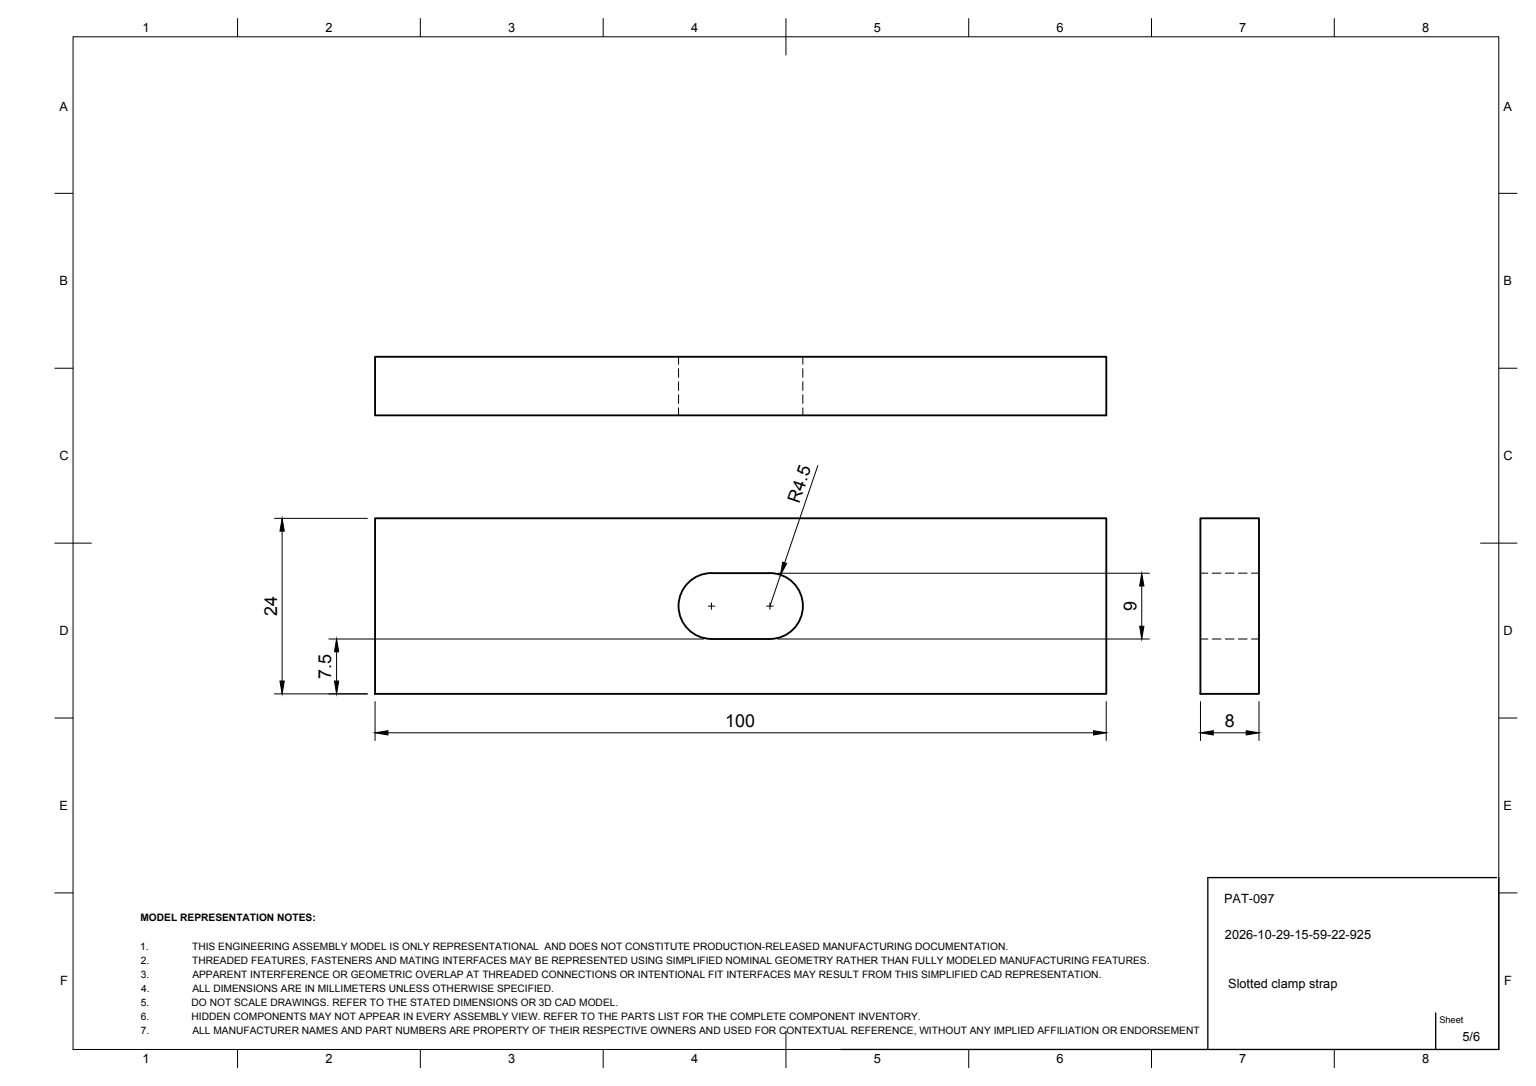
ISO-10303-21;
HEADER;
/* Generated by software containing ST-Developer
 * from STEP Tools, Inc. (www.steptools.com) 
 */

FILE_DESCRIPTION(
/* description */ ('PAT-097'),
/* implementation_level */ '2;1');

FILE_NAME(
/* name */ 'Slotted clamp strap.step',
/* time_stamp */ '2026-10-29T15:59:31-07:00',
/* author */ (''),
/* organization */ (''),
/* preprocessor_version */ 'ST-DEVELOPER v20.2',
/* originating_system */ 'Autodesk Translation Framework v15.17.0.0',
/* authorisation */ '');

FILE_SCHEMA (('AUTOMOTIVE_DESIGN { 1 0 10303 214 3 1 1 }'));
ENDSEC;

DATA;
#10=MECHANICAL_DESIGN_GEOMETRIC_PRESENTATION_REPRESENTATION('',(#78),#2768);
#64=SHAPE_REPRESENTATION_RELATIONSHIP('SRR','None',#2802,#71);
#71=ADVANCED_BREP_SHAPE_REPRESENTATION('',(#85),#2764);
#78=STYLED_ITEM('',(#2925),#85);
#85=MANIFOLD_SOLID_BREP('Body1',#1599);
#110=CYLINDRICAL_SURFACE('',#1788,0.45);
#111=CYLINDRICAL_SURFACE('',#1790,0.45);
#158=FACE_BOUND('',#403,.T.);
#159=FACE_BOUND('',#411,.T.);
#206=CIRCLE('',#1786,0.45);
#207=CIRCLE('',#1787,0.45);
#208=CIRCLE('',#1789,0.45);
#209=CIRCLE('',#1791,0.45);
#275=FACE_OUTER_BOUND('',#400,.T.);
#276=FACE_OUTER_BOUND('',#401,.T.);
#277=FACE_OUTER_BOUND('',#402,.T.);
#278=FACE_OUTER_BOUND('',#404,.T.);
#279=FACE_OUTER_BOUND('',#405,.T.);
#280=FACE_OUTER_BOUND('',#406,.T.);
#281=FACE_OUTER_BOUND('',#407,.T.);
#282=FACE_OUTER_BOUND('',#408,.T.);
#283=FACE_OUTER_BOUND('',#409,.T.);
#284=FACE_OUTER_BOUND('',#410,.T.);
#400=EDGE_LOOP('',(#1343,#1344,#1345,#1346));
#401=EDGE_LOOP('',(#1347,#1348,#1349,#1350));
#402=EDGE_LOOP('',(#1351,#1352,#1353,#1354));
#403=EDGE_LOOP('',(#1355,#1356,#1357,#1358));
#404=EDGE_LOOP('',(#1359,#1360,#1361,#1362));
#405=EDGE_LOOP('',(#1363,#1364,#1365,#1366));
#406=EDGE_LOOP('',(#1367,#1368,#1369,#1370));
#407=EDGE_LOOP('',(#1371,#1372,#1373,#1374));
#408=EDGE_LOOP('',(#1375,#1376,#1377,#1378));
#409=EDGE_LOOP('',(#1379,#1380,#1381,#1382));
#410=EDGE_LOOP('',(#1383,#1384,#1385,#1386));
#411=EDGE_LOOP('',(#1387,#1388,#1389,#1390));
#539=LINE('',#2594,#676);
#540=LINE('',#2596,#677);
#541=LINE('',#2598,#678);
#542=LINE('',#2599,#679);
#543=LINE('',#2603,#680);
#544=LINE('',#2605,#681);
#545=LINE('',#2607,#682);
#546=LINE('',#2608,#683);
#547=LINE('',#2612,#684);
#548=LINE('',#2614,#685);
#549=LINE('',#2616,#686);
#550=LINE('',#2617,#687);
#551=LINE('',#2626,#688);
#552=LINE('',#2628,#689);
#553=LINE('',#2629,#690);
#554=LINE('',#2632,#691);
#555=LINE('',#2633,#692);
#556=LINE('',#2636,#693);
#557=LINE('',#2637,#694);
#558=LINE('',#2639,#695);
#676=VECTOR('',#2148,1.);
#677=VECTOR('',#2149,1.);
#678=VECTOR('',#2150,1.);
#679=VECTOR('',#2151,1.);
#680=VECTOR('',#2154,1.);
#681=VECTOR('',#2155,1.);
#682=VECTOR('',#2156,1.);
#683=VECTOR('',#2157,1.);
#684=VECTOR('',#2160,1.);
#685=VECTOR('',#2161,1.);
#686=VECTOR('',#2162,1.);
#687=VECTOR('',#2163,1.);
#688=VECTOR('',#2178,1.);
#689=VECTOR('',#2179,1.);
#690=VECTOR('',#2180,1.);
#691=VECTOR('',#2183,1.);
#692=VECTOR('',#2184,1.);
#693=VECTOR('',#2187,1.);
#694=VECTOR('',#2188,1.);
#695=VECTOR('',#2191,1.);
#806=VERTEX_POINT('',#2592);
#807=VERTEX_POINT('',#2593);
#808=VERTEX_POINT('',#2595);
#809=VERTEX_POINT('',#2597);
#810=VERTEX_POINT('',#2601);
#811=VERTEX_POINT('',#2602);
#812=VERTEX_POINT('',#2604);
#813=VERTEX_POINT('',#2606);
#814=VERTEX_POINT('',#2610);
#815=VERTEX_POINT('',#2611);
#816=VERTEX_POINT('',#2613);
#817=VERTEX_POINT('',#2615);
#818=VERTEX_POINT('',#2625);
#819=VERTEX_POINT('',#2627);
#820=VERTEX_POINT('',#2631);
#821=VERTEX_POINT('',#2635);
#991=EDGE_CURVE('',#806,#807,#539,.T.);
#992=EDGE_CURVE('',#808,#806,#540,.T.);
#993=EDGE_CURVE('',#809,#808,#541,.T.);
#994=EDGE_CURVE('',#809,#807,#542,.T.);
#995=EDGE_CURVE('',#810,#811,#543,.T.);
#996=EDGE_CURVE('',#812,#810,#544,.T.);
#997=EDGE_CURVE('',#813,#812,#545,.T.);
#998=EDGE_CURVE('',#811,#813,#546,.T.);
#999=EDGE_CURVE('',#814,#815,#547,.T.);
#1000=EDGE_CURVE('',#816,#814,#548,.T.);
#1001=EDGE_CURVE('',#817,#816,#549,.T.);
#1002=EDGE_CURVE('',#815,#817,#550,.T.);
#1003=EDGE_CURVE('',#807,#810,#206,.T.);
#1004=EDGE_CURVE('',#811,#806,#207,.T.);
#1005=EDGE_CURVE('',#812,#809,#208,.T.);
#1006=EDGE_CURVE('',#808,#813,#209,.T.);
#1007=EDGE_CURVE('',#814,#818,#551,.T.);
#1008=EDGE_CURVE('',#819,#818,#552,.T.);
#1009=EDGE_CURVE('',#816,#819,#553,.T.);
#1010=EDGE_CURVE('',#820,#819,#554,.T.);
#1011=EDGE_CURVE('',#817,#820,#555,.T.);
#1012=EDGE_CURVE('',#821,#820,#556,.T.);
#1013=EDGE_CURVE('',#815,#821,#557,.T.);
#1014=EDGE_CURVE('',#818,#821,#558,.T.);
#1343=ORIENTED_EDGE('',*,*,#991,.F.);
#1344=ORIENTED_EDGE('',*,*,#992,.F.);
#1345=ORIENTED_EDGE('',*,*,#993,.F.);
#1346=ORIENTED_EDGE('',*,*,#994,.T.);
#1347=ORIENTED_EDGE('',*,*,#995,.F.);
#1348=ORIENTED_EDGE('',*,*,#996,.F.);
#1349=ORIENTED_EDGE('',*,*,#997,.F.);
#1350=ORIENTED_EDGE('',*,*,#998,.F.);
#1351=ORIENTED_EDGE('',*,*,#999,.F.);
#1352=ORIENTED_EDGE('',*,*,#1000,.F.);
#1353=ORIENTED_EDGE('',*,*,#1001,.F.);
#1354=ORIENTED_EDGE('',*,*,#1002,.F.);
#1355=ORIENTED_EDGE('',*,*,#991,.T.);
#1356=ORIENTED_EDGE('',*,*,#1003,.T.);
#1357=ORIENTED_EDGE('',*,*,#995,.T.);
#1358=ORIENTED_EDGE('',*,*,#1004,.T.);
#1359=ORIENTED_EDGE('',*,*,#994,.F.);
#1360=ORIENTED_EDGE('',*,*,#1005,.F.);
#1361=ORIENTED_EDGE('',*,*,#996,.T.);
#1362=ORIENTED_EDGE('',*,*,#1003,.F.);
#1363=ORIENTED_EDGE('',*,*,#992,.T.);
#1364=ORIENTED_EDGE('',*,*,#1004,.F.);
#1365=ORIENTED_EDGE('',*,*,#998,.T.);
#1366=ORIENTED_EDGE('',*,*,#1006,.F.);
#1367=ORIENTED_EDGE('',*,*,#1000,.T.);
#1368=ORIENTED_EDGE('',*,*,#1007,.T.);
#1369=ORIENTED_EDGE('',*,*,#1008,.F.);
#1370=ORIENTED_EDGE('',*,*,#1009,.F.);
#1371=ORIENTED_EDGE('',*,*,#1001,.T.);
#1372=ORIENTED_EDGE('',*,*,#1009,.T.);
#1373=ORIENTED_EDGE('',*,*,#1010,.F.);
#1374=ORIENTED_EDGE('',*,*,#1011,.F.);
#1375=ORIENTED_EDGE('',*,*,#1002,.T.);
#1376=ORIENTED_EDGE('',*,*,#1011,.T.);
#1377=ORIENTED_EDGE('',*,*,#1012,.F.);
#1378=ORIENTED_EDGE('',*,*,#1013,.F.);
#1379=ORIENTED_EDGE('',*,*,#999,.T.);
#1380=ORIENTED_EDGE('',*,*,#1013,.T.);
#1381=ORIENTED_EDGE('',*,*,#1014,.F.);
#1382=ORIENTED_EDGE('',*,*,#1007,.F.);
#1383=ORIENTED_EDGE('',*,*,#1014,.T.);
#1384=ORIENTED_EDGE('',*,*,#1012,.T.);
#1385=ORIENTED_EDGE('',*,*,#1010,.T.);
#1386=ORIENTED_EDGE('',*,*,#1008,.T.);
#1387=ORIENTED_EDGE('',*,*,#993,.T.);
#1388=ORIENTED_EDGE('',*,*,#1006,.T.);
#1389=ORIENTED_EDGE('',*,*,#997,.T.);
#1390=ORIENTED_EDGE('',*,*,#1005,.T.);
#1493=PLANE('',#1783);
#1494=PLANE('',#1784);
#1495=PLANE('',#1785);
#1496=PLANE('',#1792);
#1497=PLANE('',#1793);
#1498=PLANE('',#1794);
#1499=PLANE('',#1795);
#1500=PLANE('',#1796);
#1568=ADVANCED_FACE('',(#275),#1493,.F.);
#1569=ADVANCED_FACE('',(#276),#1494,.F.);
#1570=ADVANCED_FACE('',(#277,#158),#1495,.F.);
#1571=ADVANCED_FACE('',(#278),#110,.F.);
#1572=ADVANCED_FACE('',(#279),#111,.F.);
#1573=ADVANCED_FACE('',(#280),#1496,.T.);
#1574=ADVANCED_FACE('',(#281),#1497,.T.);
#1575=ADVANCED_FACE('',(#282),#1498,.T.);
#1576=ADVANCED_FACE('',(#283),#1499,.T.);
#1577=ADVANCED_FACE('',(#284,#159),#1500,.T.);
#1599=CLOSED_SHELL('',(#1568,#1569,#1570,#1571,#1572,#1573,#1574,#1575,
#1576,#1577));
#1782=AXIS2_PLACEMENT_3D('',#2590,#2144,#2145);
#1783=AXIS2_PLACEMENT_3D('',#2591,#2146,#2147);
#1784=AXIS2_PLACEMENT_3D('',#2600,#2152,#2153);
#1785=AXIS2_PLACEMENT_3D('',#2609,#2158,#2159);
#1786=AXIS2_PLACEMENT_3D('',#2618,#2164,#2165);
#1787=AXIS2_PLACEMENT_3D('',#2619,#2166,#2167);
#1788=AXIS2_PLACEMENT_3D('',#2620,#2168,#2169);
#1789=AXIS2_PLACEMENT_3D('',#2621,#2170,#2171);
#1790=AXIS2_PLACEMENT_3D('',#2622,#2172,#2173);
#1791=AXIS2_PLACEMENT_3D('',#2623,#2174,#2175);
#1792=AXIS2_PLACEMENT_3D('',#2624,#2176,#2177);
#1793=AXIS2_PLACEMENT_3D('',#2630,#2181,#2182);
#1794=AXIS2_PLACEMENT_3D('',#2634,#2185,#2186);
#1795=AXIS2_PLACEMENT_3D('',#2638,#2189,#2190);
#1796=AXIS2_PLACEMENT_3D('',#2640,#2192,#2193);
#2144=DIRECTION('axis',(0.,0.,1.));
#2145=DIRECTION('refdir',(1.,0.,0.));
#2146=DIRECTION('center_axis',(0.,1.,0.));
#2147=DIRECTION('ref_axis',(-1.,0.,0.));
#2148=DIRECTION('',(-1.,0.,0.));
#2149=DIRECTION('',(0.,0.,-1.));
#2150=DIRECTION('',(1.,0.,0.));
#2151=DIRECTION('',(0.,0.,-1.));
#2152=DIRECTION('center_axis',(0.,-1.,0.));
#2153=DIRECTION('ref_axis',(1.,0.,0.));
#2154=DIRECTION('',(1.,0.,0.));
#2155=DIRECTION('',(0.,0.,-1.));
#2156=DIRECTION('',(-1.,0.,0.));
#2157=DIRECTION('',(0.,0.,1.));
#2158=DIRECTION('center_axis',(0.,0.,1.));
#2159=DIRECTION('ref_axis',(1.,0.,0.));
#2160=DIRECTION('',(0.,-1.,0.));
#2161=DIRECTION('',(-1.,0.,0.));
#2162=DIRECTION('',(0.,1.,0.));
#2163=DIRECTION('',(1.,0.,0.));
#2164=DIRECTION('center_axis',(0.,0.,1.));
#2165=DIRECTION('ref_axis',(1.,0.,0.));
#2166=DIRECTION('center_axis',(0.,0.,1.));
#2167=DIRECTION('ref_axis',(1.,0.,0.));
#2168=DIRECTION('center_axis',(0.,0.,1.));
#2169=DIRECTION('ref_axis',(-1.,1.22464679914735E-16,0.));
#2170=DIRECTION('center_axis',(0.,0.,-1.));
#2171=DIRECTION('ref_axis',(1.,0.,0.));
#2172=DIRECTION('center_axis',(0.,0.,1.));
#2173=DIRECTION('ref_axis',(1.,0.,0.));
#2174=DIRECTION('center_axis',(0.,0.,-1.));
#2175=DIRECTION('ref_axis',(1.,0.,0.));
#2176=DIRECTION('center_axis',(0.,1.,0.));
#2177=DIRECTION('ref_axis',(-1.,0.,0.));
#2178=DIRECTION('',(0.,0.,1.));
#2179=DIRECTION('',(-1.,0.,0.));
#2180=DIRECTION('',(0.,0.,1.));
#2181=DIRECTION('center_axis',(1.,0.,0.));
#2182=DIRECTION('ref_axis',(0.,1.,0.));
#2183=DIRECTION('',(0.,1.,0.));
#2184=DIRECTION('',(0.,0.,1.));
#2185=DIRECTION('center_axis',(0.,-1.,0.));
#2186=DIRECTION('ref_axis',(1.,0.,0.));
#2187=DIRECTION('',(1.,0.,0.));
#2188=DIRECTION('',(0.,0.,1.));
#2189=DIRECTION('center_axis',(-1.,0.,0.));
#2190=DIRECTION('ref_axis',(0.,-1.,0.));
#2191=DIRECTION('',(0.,-1.,0.));
#2192=DIRECTION('center_axis',(0.,0.,1.));
#2193=DIRECTION('ref_axis',(1.,0.,0.));
#2590=CARTESIAN_POINT('',(0.,0.,0.));
#2591=CARTESIAN_POINT('Origin',(0.4,0.45,5.7));
#2592=CARTESIAN_POINT('',(0.4,0.45,5.8));
#2593=CARTESIAN_POINT('',(-0.4,0.45,5.8));
#2594=CARTESIAN_POINT('',(0.2,0.45,5.8));
#2595=CARTESIAN_POINT('',(0.4,0.45,6.6));
#2596=CARTESIAN_POINT('',(0.4,0.45,5.7));
#2597=CARTESIAN_POINT('',(-0.4,0.45,6.6));
#2598=CARTESIAN_POINT('',(0.2,0.45,6.6));
#2599=CARTESIAN_POINT('',(-0.4,0.45,5.7));
#2600=CARTESIAN_POINT('Origin',(-0.4,-0.45,5.7));
#2601=CARTESIAN_POINT('',(-0.4,-0.45,5.8));
#2602=CARTESIAN_POINT('',(0.4,-0.45,5.8));
#2603=CARTESIAN_POINT('',(-0.2,-0.45,5.8));
#2604=CARTESIAN_POINT('',(-0.4,-0.45,6.6));
#2605=CARTESIAN_POINT('',(-0.4,-0.45,5.7));
#2606=CARTESIAN_POINT('',(0.4,-0.45,6.6));
#2607=CARTESIAN_POINT('',(-0.2,-0.45,6.6));
#2608=CARTESIAN_POINT('',(0.4,-0.45,5.7));
#2609=CARTESIAN_POINT('Origin',(0.,0.,5.8));
#2610=CARTESIAN_POINT('',(-5.,1.2,5.8));
#2611=CARTESIAN_POINT('',(-5.,-1.2,5.8));
#2612=CARTESIAN_POINT('',(-5.,1.2,5.8));
#2613=CARTESIAN_POINT('',(5.,1.2,5.8));
#2614=CARTESIAN_POINT('',(5.,1.2,5.8));
#2615=CARTESIAN_POINT('',(5.,-1.2,5.8));
#2616=CARTESIAN_POINT('',(5.,-1.2,5.8));
#2617=CARTESIAN_POINT('',(-5.,-1.2,5.8));
#2618=CARTESIAN_POINT('Origin',(-0.4,0.,5.8));
#2619=CARTESIAN_POINT('Origin',(0.4,0.,5.8));
#2620=CARTESIAN_POINT('Origin',(-0.4,0.,5.7));
#2621=CARTESIAN_POINT('Origin',(-0.4,0.,6.6));
#2622=CARTESIAN_POINT('Origin',(0.4,0.,5.7));
#2623=CARTESIAN_POINT('Origin',(0.4,0.,6.6));
#2624=CARTESIAN_POINT('Origin',(5.,1.2,5.8));
#2625=CARTESIAN_POINT('',(-5.,1.2,6.6));
#2626=CARTESIAN_POINT('',(-5.,1.2,5.8));
#2627=CARTESIAN_POINT('',(5.,1.2,6.6));
#2628=CARTESIAN_POINT('',(5.,1.2,6.6));
#2629=CARTESIAN_POINT('',(5.,1.2,5.8));
#2630=CARTESIAN_POINT('Origin',(5.,-1.2,5.8));
#2631=CARTESIAN_POINT('',(5.,-1.2,6.6));
#2632=CARTESIAN_POINT('',(5.,-1.2,6.6));
#2633=CARTESIAN_POINT('',(5.,-1.2,5.8));
#2634=CARTESIAN_POINT('Origin',(-5.,-1.2,5.8));
#2635=CARTESIAN_POINT('',(-5.,-1.2,6.6));
#2636=CARTESIAN_POINT('',(-5.,-1.2,6.6));
#2637=CARTESIAN_POINT('',(-5.,-1.2,5.8));
#2638=CARTESIAN_POINT('Origin',(-5.,1.2,5.8));
#2639=CARTESIAN_POINT('',(-5.,1.2,6.6));
#2640=CARTESIAN_POINT('Origin',(0.,0.,6.6));
#2755=UNCERTAINTY_MEASURE_WITH_UNIT(LENGTH_MEASURE(0.001),#2769,
'DISTANCE_ACCURACY_VALUE',
'Maximum model space distance between geometric entities at asserted c
onnectivities');
#2759=UNCERTAINTY_MEASURE_WITH_UNIT(LENGTH_MEASURE(0.001),#2769,
'DISTANCE_ACCURACY_VALUE',
'Maximum model space distance between geometric entities at asserted c
onnectivities');
#2764=(
GEOMETRIC_REPRESENTATION_CONTEXT(3)
GLOBAL_UNCERTAINTY_ASSIGNED_CONTEXT((#2755))
GLOBAL_UNIT_ASSIGNED_CONTEXT((#2769,#2771,#2772))
REPRESENTATION_CONTEXT('','3D')
);
#2768=(
GEOMETRIC_REPRESENTATION_CONTEXT(3)
GLOBAL_UNCERTAINTY_ASSIGNED_CONTEXT((#2759))
GLOBAL_UNIT_ASSIGNED_CONTEXT((#2769,#2771,#2772))
REPRESENTATION_CONTEXT('','3D')
);
#2769=(
LENGTH_UNIT()
NAMED_UNIT(*)
SI_UNIT(.CENTI.,.METRE.)
);
#2771=(
NAMED_UNIT(*)
PLANE_ANGLE_UNIT()
SI_UNIT($,.RADIAN.)
);
#2772=(
NAMED_UNIT(*)
SI_UNIT($,.STERADIAN.)
SOLID_ANGLE_UNIT()
);
#2777=SHAPE_DEFINITION_REPRESENTATION(#2785,#2802);
#2785=PRODUCT_DEFINITION_SHAPE('',$,#2811);
#2802=SHAPE_REPRESENTATION('',(#1782),#2764);
#2806=PRODUCT_DEFINITION_CONTEXT('part definition',#2832,'design');
#2811=PRODUCT_DEFINITION('Slotted clamp strap',
'Slotted clamp strap',#2819,#2806);
#2819=PRODUCT_DEFINITION_FORMATION('',$,#2838);
#2832=APPLICATION_CONTEXT(
'Core Data for Automotive Mechanical Design Process');
#2833=PRODUCT_CONTEXT('part definition',#2832,'mechanical');
#2838=PRODUCT('Slotted clamp strap','Slotted clamp strap',
'Slotted clamp strap',(#2833));
#2919=COLOUR_RGB('Off White',0.89,0.88,0.83);
#2920=FILL_AREA_STYLE_COLOUR('',#2919);
#2921=FILL_AREA_STYLE('',(#2920));
#2922=SURFACE_STYLE_FILL_AREA(#2921);
#2923=SURFACE_SIDE_STYLE('',(#2922));
#2924=SURFACE_STYLE_USAGE(.BOTH.,#2923);
#2925=PRESENTATION_STYLE_ASSIGNMENT((#2924));
ENDSEC;
END-ISO-10303-21;
